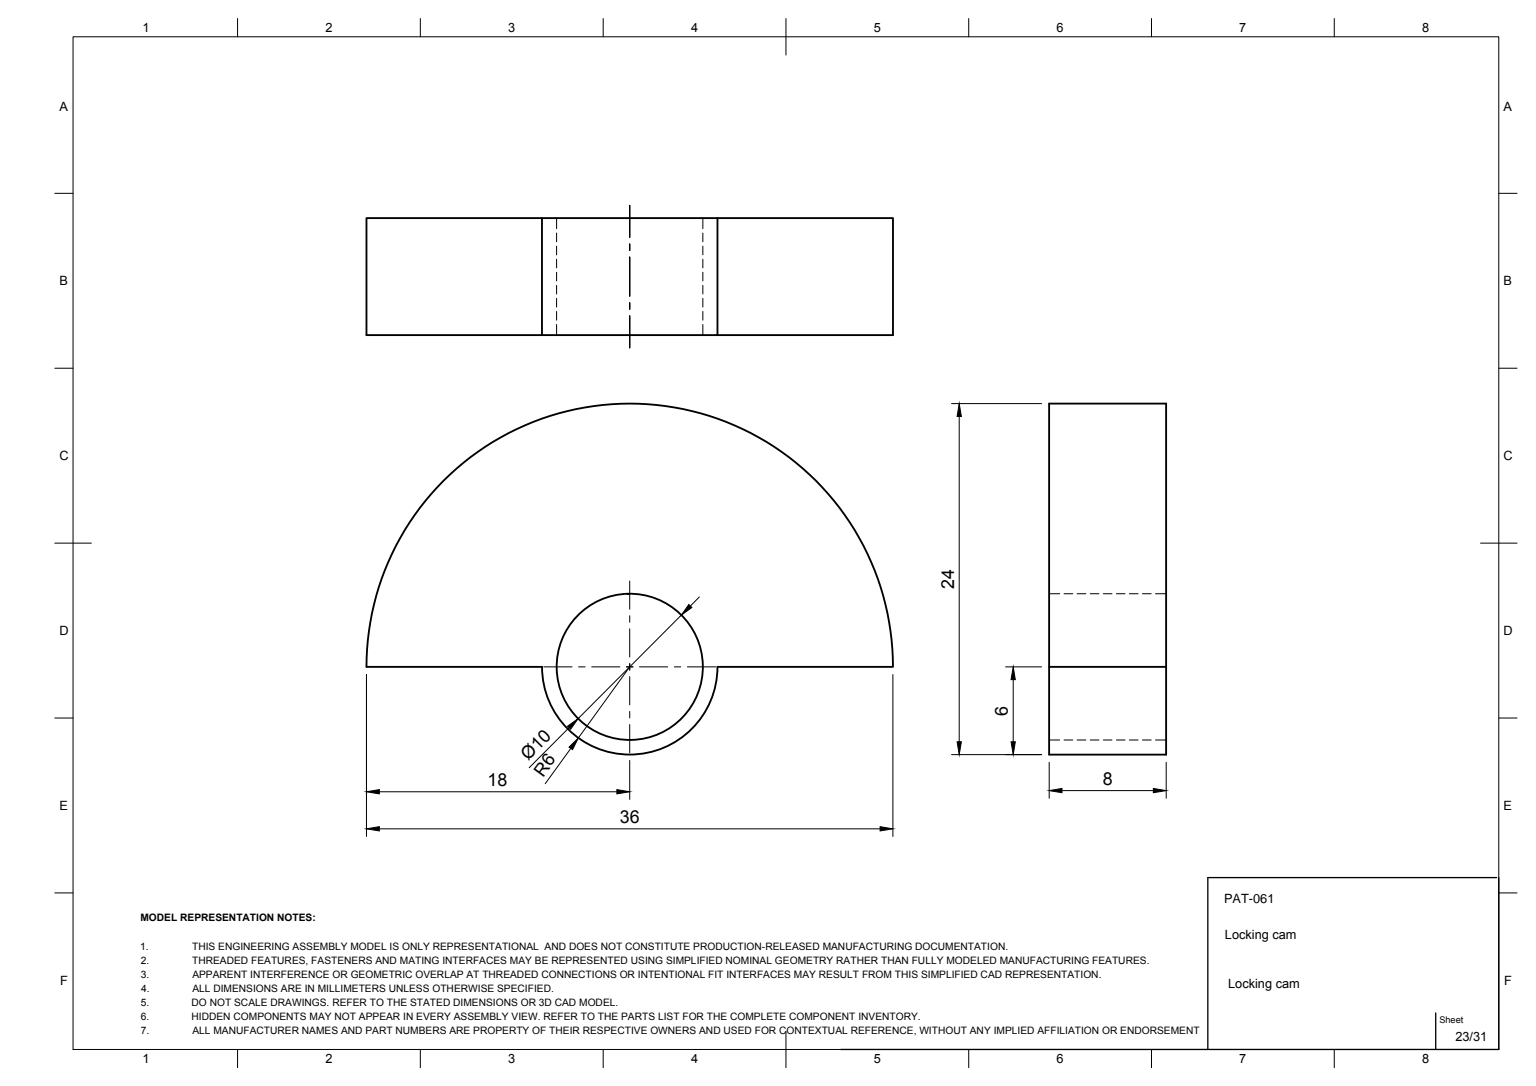
ISO-10303-21;
HEADER;
/* Generated by software containing ST-Developer
 * from STEP Tools, Inc. (www.steptools.com) 
 */

FILE_DESCRIPTION(
/* description */ ('Compact intermittent indexer'),
/* implementation_level */ '2;1');

FILE_NAME(
/* name */ 'Locking cam.step',
/* time_stamp */ '2026-10-29T16:32:17-07:00',
/* author */ (''),
/* organization */ (''),
/* preprocessor_version */ 'ST-DEVELOPER v20.2',
/* originating_system */ 'Autodesk Translation Framework v15.17.0.0',
/* authorisation */ '');

FILE_SCHEMA (('AUTOMOTIVE_DESIGN { 1 0 10303 214 3 1 1 }'));
ENDSEC;

DATA;
#10=MECHANICAL_DESIGN_GEOMETRIC_PRESENTATION_REPRESENTATION('',(#280),#10837);
#224=SHAPE_REPRESENTATION_RELATIONSHIP('SRR','None',#10960,#248);
#248=ADVANCED_BREP_SHAPE_REPRESENTATION('',(#311),#10827);
#280=STYLED_ITEM('',(#11159),#311);
#311=MANIFOLD_SOLID_BREP('Body1',#5653);
#446=FACE_BOUND('',#1293,.T.);
#447=FACE_BOUND('',#1298,.T.);
#579=PLANE('',#6409);
#580=PLANE('',#6411);
#581=PLANE('',#6412);
#582=PLANE('',#6415);
#869=FACE_OUTER_BOUND('',#1290,.T.);
#870=FACE_OUTER_BOUND('',#1291,.T.);
#871=FACE_OUTER_BOUND('',#1292,.T.);
#872=FACE_OUTER_BOUND('',#1294,.T.);
#873=FACE_OUTER_BOUND('',#1295,.T.);
#874=FACE_OUTER_BOUND('',#1296,.T.);
#875=FACE_OUTER_BOUND('',#1297,.T.);
#1290=EDGE_LOOP('',(#4606,#4607,#4608,#4609));
#1291=EDGE_LOOP('',(#4610,#4611,#4612,#4613));
#1292=EDGE_LOOP('',(#4614,#4615,#4616,#4617));
#1293=EDGE_LOOP('',(#4618));
#1294=EDGE_LOOP('',(#4619,#4620,#4621,#4622));
#1295=EDGE_LOOP('',(#4623,#4624,#4625,#4626));
#1296=EDGE_LOOP('',(#4627,#4628,#4629,#4630));
#1297=EDGE_LOOP('',(#4631,#4632,#4633,#4634));
#1298=EDGE_LOOP('',(#4635));
#1618=LINE('',#10028,#1976);
#1619=LINE('',#10033,#1977);
#1620=LINE('',#10037,#1978);
#1621=LINE('',#10041,#1979);
#1622=LINE('',#10044,#1980);
#1623=LINE('',#10047,#1981);
#1624=LINE('',#10048,#1982);
#1625=LINE('',#10051,#1983);
#1626=LINE('',#10052,#1984);
#1976=VECTOR('',#7806,0.5);
#1977=VECTOR('',#7811,1.);
#1978=VECTOR('',#7814,1.);
#1979=VECTOR('',#7819,1.);
#1980=VECTOR('',#7822,1.);
#1981=VECTOR('',#7825,1.);
#1982=VECTOR('',#7826,1.);
#1983=VECTOR('',#7829,1.);
#1984=VECTOR('',#7830,1.);
#2381=CIRCLE('',#6404,0.5);
#2382=CIRCLE('',#6405,0.5);
#2383=CIRCLE('',#6407,0.6);
#2384=CIRCLE('',#6408,0.6);
#2385=CIRCLE('',#6410,1.8);
#2386=CIRCLE('',#6414,1.8);
#2789=VERTEX_POINT('',#10025);
#2790=VERTEX_POINT('',#10027);
#2791=VERTEX_POINT('',#10031);
#2792=VERTEX_POINT('',#10032);
#2793=VERTEX_POINT('',#10034);
#2794=VERTEX_POINT('',#10036);
#2795=VERTEX_POINT('',#10040);
#2796=VERTEX_POINT('',#10042);
#2797=VERTEX_POINT('',#10046);
#2798=VERTEX_POINT('',#10050);
#3425=EDGE_CURVE('',#2789,#2789,#2381,.T.);
#3426=EDGE_CURVE('',#2789,#2790,#1618,.T.);
#3427=EDGE_CURVE('',#2790,#2790,#2382,.T.);
#3428=EDGE_CURVE('',#2791,#2792,#1619,.T.);
#3429=EDGE_CURVE('',#2793,#2791,#2383,.T.);
#3430=EDGE_CURVE('',#2794,#2793,#1620,.T.);
#3431=EDGE_CURVE('',#2794,#2792,#2384,.T.);
#3432=EDGE_CURVE('',#2794,#2795,#1621,.T.);
#3433=EDGE_CURVE('',#2796,#2795,#2385,.T.);
#3434=EDGE_CURVE('',#2796,#2792,#1622,.T.);
#3435=EDGE_CURVE('',#2797,#2793,#1623,.T.);
#3436=EDGE_CURVE('',#2795,#2797,#1624,.T.);
#3437=EDGE_CURVE('',#2798,#2796,#1625,.T.);
#3438=EDGE_CURVE('',#2791,#2798,#1626,.T.);
#3439=EDGE_CURVE('',#2798,#2797,#2386,.T.);
#4606=ORIENTED_EDGE('',*,*,#3425,.F.);
#4607=ORIENTED_EDGE('',*,*,#3426,.T.);
#4608=ORIENTED_EDGE('',*,*,#3427,.F.);
#4609=ORIENTED_EDGE('',*,*,#3426,.F.);
#4610=ORIENTED_EDGE('',*,*,#3428,.F.);
#4611=ORIENTED_EDGE('',*,*,#3429,.F.);
#4612=ORIENTED_EDGE('',*,*,#3430,.F.);
#4613=ORIENTED_EDGE('',*,*,#3431,.T.);
#4614=ORIENTED_EDGE('',*,*,#3432,.T.);
#4615=ORIENTED_EDGE('',*,*,#3433,.F.);
#4616=ORIENTED_EDGE('',*,*,#3434,.T.);
#4617=ORIENTED_EDGE('',*,*,#3431,.F.);
#4618=ORIENTED_EDGE('',*,*,#3425,.T.);
#4619=ORIENTED_EDGE('',*,*,#3430,.T.);
#4620=ORIENTED_EDGE('',*,*,#3435,.F.);
#4621=ORIENTED_EDGE('',*,*,#3436,.F.);
#4622=ORIENTED_EDGE('',*,*,#3432,.F.);
#4623=ORIENTED_EDGE('',*,*,#3428,.T.);
#4624=ORIENTED_EDGE('',*,*,#3434,.F.);
#4625=ORIENTED_EDGE('',*,*,#3437,.F.);
#4626=ORIENTED_EDGE('',*,*,#3438,.F.);
#4627=ORIENTED_EDGE('',*,*,#3437,.T.);
#4628=ORIENTED_EDGE('',*,*,#3433,.T.);
#4629=ORIENTED_EDGE('',*,*,#3436,.T.);
#4630=ORIENTED_EDGE('',*,*,#3439,.F.);
#4631=ORIENTED_EDGE('',*,*,#3438,.T.);
#4632=ORIENTED_EDGE('',*,*,#3439,.T.);
#4633=ORIENTED_EDGE('',*,*,#3435,.T.);
#4634=ORIENTED_EDGE('',*,*,#3429,.T.);
#4635=ORIENTED_EDGE('',*,*,#3427,.T.);
#5255=CYLINDRICAL_SURFACE('',#6403,0.5);
#5256=CYLINDRICAL_SURFACE('',#6406,0.6);
#5257=CYLINDRICAL_SURFACE('',#6413,1.8);
#5512=ADVANCED_FACE('',(#869),#5255,.F.);
#5513=ADVANCED_FACE('',(#870),#5256,.T.);
#5514=ADVANCED_FACE('',(#871,#446),#579,.F.);
#5515=ADVANCED_FACE('',(#872),#580,.F.);
#5516=ADVANCED_FACE('',(#873),#581,.F.);
#5517=ADVANCED_FACE('',(#874),#5257,.T.);
#5518=ADVANCED_FACE('',(#875,#447),#582,.T.);
#5653=CLOSED_SHELL('',(#5512,#5513,#5514,#5515,#5516,#5517,#5518));
#6402=AXIS2_PLACEMENT_3D('',#10023,#7800,#7801);
#6403=AXIS2_PLACEMENT_3D('',#10024,#7802,#7803);
#6404=AXIS2_PLACEMENT_3D('',#10026,#7804,#7805);
#6405=AXIS2_PLACEMENT_3D('',#10029,#7807,#7808);
#6406=AXIS2_PLACEMENT_3D('',#10030,#7809,#7810);
#6407=AXIS2_PLACEMENT_3D('',#10035,#7812,#7813);
#6408=AXIS2_PLACEMENT_3D('',#10038,#7815,#7816);
#6409=AXIS2_PLACEMENT_3D('',#10039,#7817,#7818);
#6410=AXIS2_PLACEMENT_3D('',#10043,#7820,#7821);
#6411=AXIS2_PLACEMENT_3D('',#10045,#7823,#7824);
#6412=AXIS2_PLACEMENT_3D('',#10049,#7827,#7828);
#6413=AXIS2_PLACEMENT_3D('',#10053,#7831,#7832);
#6414=AXIS2_PLACEMENT_3D('',#10054,#7833,#7834);
#6415=AXIS2_PLACEMENT_3D('',#10055,#7835,#7836);
#7800=DIRECTION('axis',(0.,0.,1.));
#7801=DIRECTION('refdir',(1.,0.,0.));
#7802=DIRECTION('center_axis',(0.,0.,1.));
#7803=DIRECTION('ref_axis',(1.,0.,0.));
#7804=DIRECTION('center_axis',(0.,0.,1.));
#7805=DIRECTION('ref_axis',(1.,0.,0.));
#7806=DIRECTION('',(0.,0.,1.));
#7807=DIRECTION('center_axis',(0.,0.,-1.));
#7808=DIRECTION('ref_axis',(1.,0.,0.));
#7809=DIRECTION('center_axis',(0.,0.,1.));
#7810=DIRECTION('ref_axis',(1.,0.,0.));
#7811=DIRECTION('',(0.,0.,-1.));
#7812=DIRECTION('center_axis',(0.,0.,1.));
#7813=DIRECTION('ref_axis',(1.,0.,0.));
#7814=DIRECTION('',(0.,0.,1.));
#7815=DIRECTION('center_axis',(0.,0.,1.));
#7816=DIRECTION('ref_axis',(1.,0.,0.));
#7817=DIRECTION('center_axis',(0.,0.,1.));
#7818=DIRECTION('ref_axis',(1.,0.,0.));
#7819=DIRECTION('',(0.,-1.,0.));
#7820=DIRECTION('center_axis',(0.,0.,1.));
#7821=DIRECTION('ref_axis',(1.,0.,0.));
#7822=DIRECTION('',(0.,-1.,0.));
#7823=DIRECTION('center_axis',(-1.,0.,0.));
#7824=DIRECTION('ref_axis',(0.,-1.,0.));
#7825=DIRECTION('',(0.,1.,0.));
#7826=DIRECTION('',(0.,0.,1.));
#7827=DIRECTION('center_axis',(-1.,0.,0.));
#7828=DIRECTION('ref_axis',(0.,-1.,0.));
#7829=DIRECTION('',(0.,0.,-1.));
#7830=DIRECTION('',(0.,1.,0.));
#7831=DIRECTION('center_axis',(0.,0.,1.));
#7832=DIRECTION('ref_axis',(-1.,1.22464679914735E-16,0.));
#7833=DIRECTION('center_axis',(0.,0.,1.));
#7834=DIRECTION('ref_axis',(1.,0.,0.));
#7835=DIRECTION('center_axis',(0.,0.,1.));
#7836=DIRECTION('ref_axis',(1.,0.,0.));
#10023=CARTESIAN_POINT('',(0.,0.,0.));
#10024=CARTESIAN_POINT('Origin',(0.,0.,5.9));
#10025=CARTESIAN_POINT('',(-0.5,-6.12323399573677E-17,6.));
#10026=CARTESIAN_POINT('Origin',(0.,0.,6.));
#10027=CARTESIAN_POINT('',(-0.5,6.12323399573677E-17,6.8));
#10028=CARTESIAN_POINT('',(-0.5,-6.12323399573677E-17,5.9));
#10029=CARTESIAN_POINT('Origin',(0.,0.,6.8));
#10030=CARTESIAN_POINT('Origin',(0.,0.,6.));
#10031=CARTESIAN_POINT('',(0.,0.6,6.8));
#10032=CARTESIAN_POINT('',(0.,0.6,6.));
#10033=CARTESIAN_POINT('',(0.,0.6,6.));
#10034=CARTESIAN_POINT('',(0.,-0.6,6.8));
#10035=CARTESIAN_POINT('Origin',(0.,0.,6.8));
#10036=CARTESIAN_POINT('',(0.,-0.6,6.));
#10037=CARTESIAN_POINT('',(0.,-0.6,6.));
#10038=CARTESIAN_POINT('Origin',(0.,0.,6.));
#10039=CARTESIAN_POINT('Origin',(0.,0.,6.));
#10040=CARTESIAN_POINT('',(0.,-1.8,6.));
#10041=CARTESIAN_POINT('',(0.,0.95,6.));
#10042=CARTESIAN_POINT('',(0.,1.8,6.));
#10043=CARTESIAN_POINT('Origin',(0.,0.,6.));
#10044=CARTESIAN_POINT('',(0.,0.95,6.));
#10045=CARTESIAN_POINT('Origin',(0.,1.9,5.9));
#10046=CARTESIAN_POINT('',(0.,-1.8,6.8));
#10047=CARTESIAN_POINT('',(0.,0.95,6.8));
#10048=CARTESIAN_POINT('',(0.,-1.8,6.));
#10049=CARTESIAN_POINT('Origin',(0.,1.9,5.9));
#10050=CARTESIAN_POINT('',(0.,1.8,6.8));
#10051=CARTESIAN_POINT('',(0.,1.8,6.));
#10052=CARTESIAN_POINT('',(0.,0.95,6.8));
#10053=CARTESIAN_POINT('Origin',(0.,0.,6.));
#10054=CARTESIAN_POINT('Origin',(0.,0.,6.8));
#10055=CARTESIAN_POINT('Origin',(0.,0.,6.8));
#10797=UNCERTAINTY_MEASURE_WITH_UNIT(LENGTH_MEASURE(0.001),#10838,
'DISTANCE_ACCURACY_VALUE',
'Maximum model space distance between geometric entities at asserted c
onnectivities');
#10807=UNCERTAINTY_MEASURE_WITH_UNIT(LENGTH_MEASURE(0.001),#10838,
'DISTANCE_ACCURACY_VALUE',
'Maximum model space distance between geometric entities at asserted c
onnectivities');
#10827=(
GEOMETRIC_REPRESENTATION_CONTEXT(3)
GLOBAL_UNCERTAINTY_ASSIGNED_CONTEXT((#10797))
GLOBAL_UNIT_ASSIGNED_CONTEXT((#10838,#10840,#10841))
REPRESENTATION_CONTEXT('','3D')
);
#10837=(
GEOMETRIC_REPRESENTATION_CONTEXT(3)
GLOBAL_UNCERTAINTY_ASSIGNED_CONTEXT((#10807))
GLOBAL_UNIT_ASSIGNED_CONTEXT((#10838,#10840,#10841))
REPRESENTATION_CONTEXT('','3D')
);
#10838=(
LENGTH_UNIT()
NAMED_UNIT(*)
SI_UNIT(.CENTI.,.METRE.)
);
#10840=(
NAMED_UNIT(*)
PLANE_ANGLE_UNIT()
SI_UNIT($,.RADIAN.)
);
#10841=(
NAMED_UNIT(*)
SI_UNIT($,.STERADIAN.)
SOLID_ANGLE_UNIT()
);
#10861=SHAPE_DEFINITION_REPRESENTATION(#10895,#10960);
#10895=PRODUCT_DEFINITION_SHAPE('',$,#10990);
#10960=SHAPE_REPRESENTATION('',(#6402),#10827);
#10970=PRODUCT_DEFINITION_CONTEXT('part definition',#11059,'design');
#10990=PRODUCT_DEFINITION('Locking cam','Locking cam',#11019,#10970);
#11019=PRODUCT_DEFINITION_FORMATION('',$,#11080);
#11059=APPLICATION_CONTEXT(
'Core Data for Automotive Mechanical Design Process');
#11060=PRODUCT_CONTEXT('part definition',#11059,'mechanical');
#11080=PRODUCT('Locking cam','Locking cam','Locking cam',(#11060));
#11153=COLOUR_RGB('Sky Blue',0.24,0.69,0.87);
#11154=FILL_AREA_STYLE_COLOUR('',#11153);
#11155=FILL_AREA_STYLE('',(#11154));
#11156=SURFACE_STYLE_FILL_AREA(#11155);
#11157=SURFACE_SIDE_STYLE('',(#11156));
#11158=SURFACE_STYLE_USAGE(.BOTH.,#11157);
#11159=PRESENTATION_STYLE_ASSIGNMENT((#11158));
ENDSEC;
END-ISO-10303-21;
